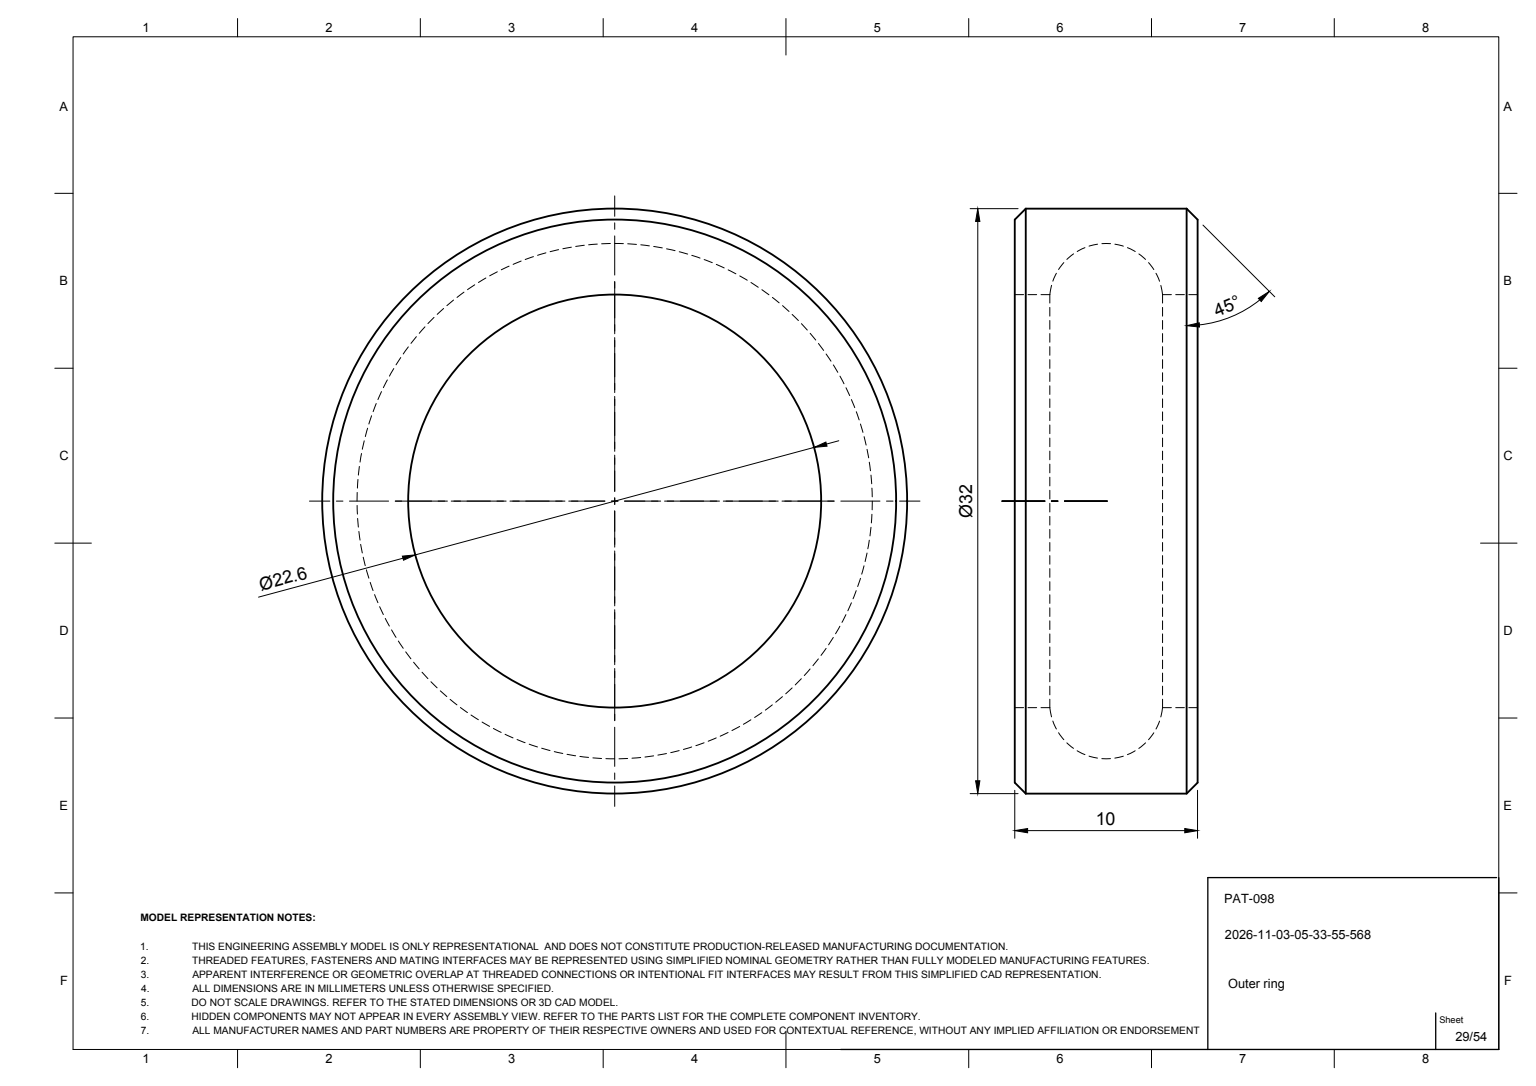
ISO-10303-21;
HEADER;
/* Generated by software containing ST-Developer
 * from STEP Tools, Inc. (www.steptools.com) 
 */

FILE_DESCRIPTION(
/* description */ ('Spring compression tester'),
/* implementation_level */ '2;1');

FILE_NAME(
/* name */ 'Outer ring.step',
/* time_stamp */ '2026-10-28T03:24:11-07:00',
/* author */ (''),
/* organization */ (''),
/* preprocessor_version */ 'ST-DEVELOPER v20.2',
/* originating_system */ 'Autodesk Translation Framework v15.17.0.0',
/* authorisation */ '');

FILE_SCHEMA (('AUTOMOTIVE_DESIGN { 1 0 10303 214 3 1 1 }'));
ENDSEC;

DATA;
#10=MECHANICAL_DESIGN_GEOMETRIC_PRESENTATION_REPRESENTATION('',(#1128),#43521);
#928=TOROIDAL_SURFACE('',#20014,1.1,0.309556);
#952=CONICAL_SURFACE('',#20025,1.57,0.785398163397449);
#953=CONICAL_SURFACE('',#20029,1.57,0.785398163397449);
#1008=SHAPE_REPRESENTATION_RELATIONSHIP('SRR','None',#43821,#1068);
#1068=ADVANCED_BREP_SHAPE_REPRESENTATION('',(#1202),#43481);
#1128=STYLED_ITEM('',(#44202),#1202);
#1202=MANIFOLD_SOLID_BREP('Body1',#18566);
#1452=FACE_BOUND('',#3859,.T.);
#1453=FACE_BOUND('',#3864,.T.);
#1890=PLANE('',#20022);
#1891=PLANE('',#20031);
#2604=FACE_OUTER_BOUND('',#3856,.T.);
#2605=FACE_OUTER_BOUND('',#3857,.T.);
#2606=FACE_OUTER_BOUND('',#3858,.T.);
#2607=FACE_OUTER_BOUND('',#3860,.T.);
#2608=FACE_OUTER_BOUND('',#3861,.T.);
#2609=FACE_OUTER_BOUND('',#3862,.T.);
#2610=FACE_OUTER_BOUND('',#3863,.T.);
#2611=FACE_OUTER_BOUND('',#3865,.T.);
#3856=EDGE_LOOP('',(#14153,#14154,#14155,#14156,#14157,#14158));
#3857=EDGE_LOOP('',(#14159,#14160,#14161,#14162,#14163));
#3858=EDGE_LOOP('',(#14164));
#3859=EDGE_LOOP('',(#14165));
#3860=EDGE_LOOP('',(#14166,#14167,#14168,#14169));
#3861=EDGE_LOOP('',(#14170,#14171,#14172,#14173));
#3862=EDGE_LOOP('',(#14174,#14175,#14176,#14177));
#3863=EDGE_LOOP('',(#14178));
#3864=EDGE_LOOP('',(#14179));
#3865=EDGE_LOOP('',(#14180,#14181,#14182,#14183,#14184));
#5306=LINE('',#28538,#6738);
#5307=LINE('',#28547,#6739);
#5308=LINE('',#28551,#6740);
#5309=LINE('',#28555,#6741);
#5310=LINE('',#28558,#6742);
#6738=VECTOR('',#23372,1.129765);
#6739=VECTOR('',#23383,1.57);
#6740=VECTOR('',#23388,1.6);
#6741=VECTOR('',#23393,1.57);
#6742=VECTOR('',#23398,1.129765);
#7738=CIRCLE('',#20015,1.129765);
#7739=CIRCLE('',#20016,1.129765);
#7740=CIRCLE('',#20017,0.309556);
#7741=CIRCLE('',#20018,1.129765);
#7742=CIRCLE('',#20019,1.129765);
#7743=CIRCLE('',#20021,1.129765);
#7744=CIRCLE('',#20023,1.54);
#7745=CIRCLE('',#20024,1.129765);
#7746=CIRCLE('',#20026,1.6);
#7747=CIRCLE('',#20028,1.6);
#7748=CIRCLE('',#20030,1.54);
#8779=VERTEX_POINT('',#28526);
#8780=VERTEX_POINT('',#28527);
#8781=VERTEX_POINT('',#28530);
#8782=VERTEX_POINT('',#28532);
#8783=VERTEX_POINT('',#28536);
#8784=VERTEX_POINT('',#28540);
#8785=VERTEX_POINT('',#28542);
#8786=VERTEX_POINT('',#28545);
#8787=VERTEX_POINT('',#28549);
#8788=VERTEX_POINT('',#28553);
#10741=EDGE_CURVE('',#8779,#8780,#7738,.T.);
#10742=EDGE_CURVE('',#8780,#8779,#7739,.T.);
#10743=EDGE_CURVE('',#8780,#8781,#7740,.T.);
#10744=EDGE_CURVE('',#8782,#8781,#7741,.T.);
#10745=EDGE_CURVE('',#8781,#8782,#7742,.T.);
#10746=EDGE_CURVE('',#8783,#8783,#7743,.T.);
#10747=EDGE_CURVE('',#8783,#8782,#5306,.T.);
#10748=EDGE_CURVE('',#8784,#8784,#7744,.T.);
#10749=EDGE_CURVE('',#8785,#8785,#7745,.T.);
#10750=EDGE_CURVE('',#8786,#8786,#7746,.T.);
#10751=EDGE_CURVE('',#8786,#8784,#5307,.T.);
#10752=EDGE_CURVE('',#8787,#8787,#7747,.T.);
#10753=EDGE_CURVE('',#8787,#8786,#5308,.T.);
#10754=EDGE_CURVE('',#8788,#8788,#7748,.T.);
#10755=EDGE_CURVE('',#8788,#8787,#5309,.T.);
#10756=EDGE_CURVE('',#8779,#8785,#5310,.T.);
#14153=ORIENTED_EDGE('',*,*,#10741,.F.);
#14154=ORIENTED_EDGE('',*,*,#10742,.F.);
#14155=ORIENTED_EDGE('',*,*,#10743,.T.);
#14156=ORIENTED_EDGE('',*,*,#10744,.F.);
#14157=ORIENTED_EDGE('',*,*,#10745,.F.);
#14158=ORIENTED_EDGE('',*,*,#10743,.F.);
#14159=ORIENTED_EDGE('',*,*,#10746,.T.);
#14160=ORIENTED_EDGE('',*,*,#10747,.T.);
#14161=ORIENTED_EDGE('',*,*,#10744,.T.);
#14162=ORIENTED_EDGE('',*,*,#10745,.T.);
#14163=ORIENTED_EDGE('',*,*,#10747,.F.);
#14164=ORIENTED_EDGE('',*,*,#10748,.F.);
#14165=ORIENTED_EDGE('',*,*,#10749,.T.);
#14166=ORIENTED_EDGE('',*,*,#10750,.F.);
#14167=ORIENTED_EDGE('',*,*,#10751,.T.);
#14168=ORIENTED_EDGE('',*,*,#10748,.T.);
#14169=ORIENTED_EDGE('',*,*,#10751,.F.);
#14170=ORIENTED_EDGE('',*,*,#10752,.F.);
#14171=ORIENTED_EDGE('',*,*,#10753,.T.);
#14172=ORIENTED_EDGE('',*,*,#10750,.T.);
#14173=ORIENTED_EDGE('',*,*,#10753,.F.);
#14174=ORIENTED_EDGE('',*,*,#10754,.F.);
#14175=ORIENTED_EDGE('',*,*,#10755,.T.);
#14176=ORIENTED_EDGE('',*,*,#10752,.T.);
#14177=ORIENTED_EDGE('',*,*,#10755,.F.);
#14178=ORIENTED_EDGE('',*,*,#10754,.T.);
#14179=ORIENTED_EDGE('',*,*,#10746,.F.);
#14180=ORIENTED_EDGE('',*,*,#10741,.T.);
#14181=ORIENTED_EDGE('',*,*,#10742,.T.);
#14182=ORIENTED_EDGE('',*,*,#10756,.T.);
#14183=ORIENTED_EDGE('',*,*,#10749,.F.);
#14184=ORIENTED_EDGE('',*,*,#10756,.F.);
#17230=CYLINDRICAL_SURFACE('',#20020,1.129765);
#17231=CYLINDRICAL_SURFACE('',#20027,1.6);
#17232=CYLINDRICAL_SURFACE('',#20032,1.129765);
#17928=ADVANCED_FACE('',(#2604),#928,.F.);
#17929=ADVANCED_FACE('',(#2605),#17230,.F.);
#17930=ADVANCED_FACE('',(#2606,#1452),#1890,.T.);
#17931=ADVANCED_FACE('',(#2607),#952,.T.);
#17932=ADVANCED_FACE('',(#2608),#17231,.T.);
#17933=ADVANCED_FACE('',(#2609),#953,.T.);
#17934=ADVANCED_FACE('',(#2610,#1453),#1891,.T.);
#17935=ADVANCED_FACE('',(#2611),#17232,.F.);
#18566=CLOSED_SHELL('',(#17928,#17929,#17930,#17931,#17932,#17933,#17934,
#17935));
#20013=AXIS2_PLACEMENT_3D('',#28524,#23354,#23355);
#20014=AXIS2_PLACEMENT_3D('',#28525,#23356,#23357);
#20015=AXIS2_PLACEMENT_3D('',#28528,#23358,#23359);
#20016=AXIS2_PLACEMENT_3D('',#28529,#23360,#23361);
#20017=AXIS2_PLACEMENT_3D('',#28531,#23362,#23363);
#20018=AXIS2_PLACEMENT_3D('',#28533,#23364,#23365);
#20019=AXIS2_PLACEMENT_3D('',#28534,#23366,#23367);
#20020=AXIS2_PLACEMENT_3D('',#28535,#23368,#23369);
#20021=AXIS2_PLACEMENT_3D('',#28537,#23370,#23371);
#20022=AXIS2_PLACEMENT_3D('',#28539,#23373,#23374);
#20023=AXIS2_PLACEMENT_3D('',#28541,#23375,#23376);
#20024=AXIS2_PLACEMENT_3D('',#28543,#23377,#23378);
#20025=AXIS2_PLACEMENT_3D('',#28544,#23379,#23380);
#20026=AXIS2_PLACEMENT_3D('',#28546,#23381,#23382);
#20027=AXIS2_PLACEMENT_3D('',#28548,#23384,#23385);
#20028=AXIS2_PLACEMENT_3D('',#28550,#23386,#23387);
#20029=AXIS2_PLACEMENT_3D('',#28552,#23389,#23390);
#20030=AXIS2_PLACEMENT_3D('',#28554,#23391,#23392);
#20031=AXIS2_PLACEMENT_3D('',#28556,#23394,#23395);
#20032=AXIS2_PLACEMENT_3D('',#28557,#23396,#23397);
#23354=DIRECTION('axis',(0.,0.,1.));
#23355=DIRECTION('refdir',(1.,0.,0.));
#23356=DIRECTION('center_axis',(0.,-1.,0.));
#23357=DIRECTION('ref_axis',(0.,0.,-1.));
#23358=DIRECTION('center_axis',(0.,-1.,0.));
#23359=DIRECTION('ref_axis',(1.,0.,0.));
#23360=DIRECTION('center_axis',(0.,-1.,0.));
#23361=DIRECTION('ref_axis',(1.,0.,0.));
#23362=DIRECTION('center_axis',(1.,0.,1.22464679914735E-16));
#23363=DIRECTION('ref_axis',(-1.22464679914735E-16,0.,1.));
#23364=DIRECTION('center_axis',(0.,1.,0.));
#23365=DIRECTION('ref_axis',(1.,0.,0.));
#23366=DIRECTION('center_axis',(0.,1.,0.));
#23367=DIRECTION('ref_axis',(1.,0.,0.));
#23368=DIRECTION('center_axis',(0.,-1.,0.));
#23369=DIRECTION('ref_axis',(1.,0.,0.));
#23370=DIRECTION('center_axis',(0.,-1.,0.));
#23371=DIRECTION('ref_axis',(1.,0.,0.));
#23372=DIRECTION('',(0.,1.,0.));
#23373=DIRECTION('center_axis',(0.,1.,0.));
#23374=DIRECTION('ref_axis',(0.,0.,1.));
#23375=DIRECTION('center_axis',(0.,-1.,0.));
#23376=DIRECTION('ref_axis',(1.,0.,0.));
#23377=DIRECTION('center_axis',(0.,-1.,0.));
#23378=DIRECTION('ref_axis',(1.,0.,0.));
#23379=DIRECTION('center_axis',(0.,-1.,0.));
#23380=DIRECTION('ref_axis',(1.,0.,0.));
#23381=DIRECTION('center_axis',(0.,-1.,0.));
#23382=DIRECTION('ref_axis',(1.,0.,0.));
#23383=DIRECTION('',(0.707106781186548,0.707106781186547,8.65956056235494E-17));
#23384=DIRECTION('center_axis',(0.,-1.,0.));
#23385=DIRECTION('ref_axis',(1.,0.,0.));
#23386=DIRECTION('center_axis',(0.,-1.,0.));
#23387=DIRECTION('ref_axis',(1.,0.,0.));
#23388=DIRECTION('',(0.,1.,0.));
#23389=DIRECTION('center_axis',(0.,1.,0.));
#23390=DIRECTION('ref_axis',(1.,0.,0.));
#23391=DIRECTION('center_axis',(0.,-1.,0.));
#23392=DIRECTION('ref_axis',(1.,0.,0.));
#23393=DIRECTION('',(-0.707106781186548,0.707106781186547,-8.65956056235494E-17));
#23394=DIRECTION('center_axis',(0.,-1.,0.));
#23395=DIRECTION('ref_axis',(0.,0.,-1.));
#23396=DIRECTION('center_axis',(0.,-1.,0.));
#23397=DIRECTION('ref_axis',(1.,0.,0.));
#23398=DIRECTION('',(0.,1.,0.));
#28524=CARTESIAN_POINT('',(0.,0.,0.));
#28525=CARTESIAN_POINT('Origin',(0.,0.,0.));
#28526=CARTESIAN_POINT('',(-1.129765,0.308121667383195,-1.38356309103871E-16));
#28527=CARTESIAN_POINT('',(-1.38356309103871E-16,0.308121667383195,1.129765));
#28528=CARTESIAN_POINT('Origin',(0.,0.308121667383195,0.));
#28529=CARTESIAN_POINT('Origin',(0.,0.308121667383195,0.));
#28530=CARTESIAN_POINT('',(-1.38356309103871E-16,-0.308121667383195,1.129765));
#28531=CARTESIAN_POINT('Origin',(-1.34711147906209E-16,0.,1.1));
#28532=CARTESIAN_POINT('',(-1.129765,-0.308121667383195,1.38356309103871E-16));
#28533=CARTESIAN_POINT('Origin',(0.,-0.308121667383195,0.));
#28534=CARTESIAN_POINT('Origin',(0.,-0.308121667383195,0.));
#28535=CARTESIAN_POINT('Origin',(0.,0.,0.));
#28536=CARTESIAN_POINT('',(-1.129765,-0.5,-1.38356309103871E-16));
#28537=CARTESIAN_POINT('Origin',(0.,-0.5,0.));
#28538=CARTESIAN_POINT('',(-1.129765,0.,-1.38356309103871E-16));
#28539=CARTESIAN_POINT('Origin',(1.54,0.5,0.));
#28540=CARTESIAN_POINT('',(-1.54,0.5,-1.88595607068692E-16));
#28541=CARTESIAN_POINT('Origin',(0.,0.5,0.));
#28542=CARTESIAN_POINT('',(-1.129765,0.5,-1.38356309103871E-16));
#28543=CARTESIAN_POINT('Origin',(0.,0.5,0.));
#28544=CARTESIAN_POINT('Origin',(0.,0.47,0.));
#28545=CARTESIAN_POINT('',(-1.6,0.44,-1.95943487863577E-16));
#28546=CARTESIAN_POINT('Origin',(0.,0.44,0.));
#28547=CARTESIAN_POINT('',(-1.57,0.47,-1.92269547466134E-16));
#28548=CARTESIAN_POINT('Origin',(0.,0.,0.));
#28549=CARTESIAN_POINT('',(-1.6,-0.44,-1.95943487863577E-16));
#28550=CARTESIAN_POINT('Origin',(0.,-0.44,0.));
#28551=CARTESIAN_POINT('',(-1.6,0.,-1.95943487863577E-16));
#28552=CARTESIAN_POINT('Origin',(0.,-0.47,0.));
#28553=CARTESIAN_POINT('',(-1.54,-0.5,-1.88595607068692E-16));
#28554=CARTESIAN_POINT('Origin',(0.,-0.5,0.));
#28555=CARTESIAN_POINT('',(-1.57,-0.47,-1.92269547466134E-16));
#28556=CARTESIAN_POINT('Origin',(1.129765,-0.5,0.));
#28557=CARTESIAN_POINT('Origin',(0.,0.,0.));
#28558=CARTESIAN_POINT('',(-1.129765,0.,-1.38356309103871E-16));
#43413=UNCERTAINTY_MEASURE_WITH_UNIT(LENGTH_MEASURE(0.001),#43522,
'DISTANCE_ACCURACY_VALUE',
'Maximum model space distance between geometric entities at asserted c
onnectivities');
#43453=UNCERTAINTY_MEASURE_WITH_UNIT(LENGTH_MEASURE(0.001),#43522,
'DISTANCE_ACCURACY_VALUE',
'Maximum model space distance between geometric entities at asserted c
onnectivities');
#43481=(
GEOMETRIC_REPRESENTATION_CONTEXT(3)
GLOBAL_UNCERTAINTY_ASSIGNED_CONTEXT((#43413))
GLOBAL_UNIT_ASSIGNED_CONTEXT((#43522,#43524,#43525))
REPRESENTATION_CONTEXT('','3D')
);
#43521=(
GEOMETRIC_REPRESENTATION_CONTEXT(3)
GLOBAL_UNCERTAINTY_ASSIGNED_CONTEXT((#43453))
GLOBAL_UNIT_ASSIGNED_CONTEXT((#43522,#43524,#43525))
REPRESENTATION_CONTEXT('','3D')
);
#43522=(
LENGTH_UNIT()
NAMED_UNIT(*)
SI_UNIT(.CENTI.,.METRE.)
);
#43524=(
NAMED_UNIT(*)
PLANE_ANGLE_UNIT()
SI_UNIT($,.RADIAN.)
);
#43525=(
NAMED_UNIT(*)
SI_UNIT($,.STERADIAN.)
SOLID_ANGLE_UNIT()
);
#43553=SHAPE_DEFINITION_REPRESENTATION(#43620,#43821);
#43620=PRODUCT_DEFINITION_SHAPE('',$,#43889);
#43821=SHAPE_REPRESENTATION('',(#20013),#43481);
#43861=PRODUCT_DEFINITION_CONTEXT('part definition',#44064,'design');
#43889=PRODUCT_DEFINITION('Outer ring','Outer ring',#43956,#43861);
#43956=PRODUCT_DEFINITION_FORMATION('',$,#44093);
#44064=APPLICATION_CONTEXT(
'Core Data for Automotive Mechanical Design Process');
#44065=PRODUCT_CONTEXT('part definition',#44064,'mechanical');
#44093=PRODUCT('Outer ring','Outer ring','Outer ring',(#44065));
#44196=COLOUR_RGB('Grey',0.48,0.52,0.57);
#44197=FILL_AREA_STYLE_COLOUR('',#44196);
#44198=FILL_AREA_STYLE('',(#44197));
#44199=SURFACE_STYLE_FILL_AREA(#44198);
#44200=SURFACE_SIDE_STYLE('',(#44199));
#44201=SURFACE_STYLE_USAGE(.BOTH.,#44200);
#44202=PRESENTATION_STYLE_ASSIGNMENT((#44201));
ENDSEC;
END-ISO-10303-21;
